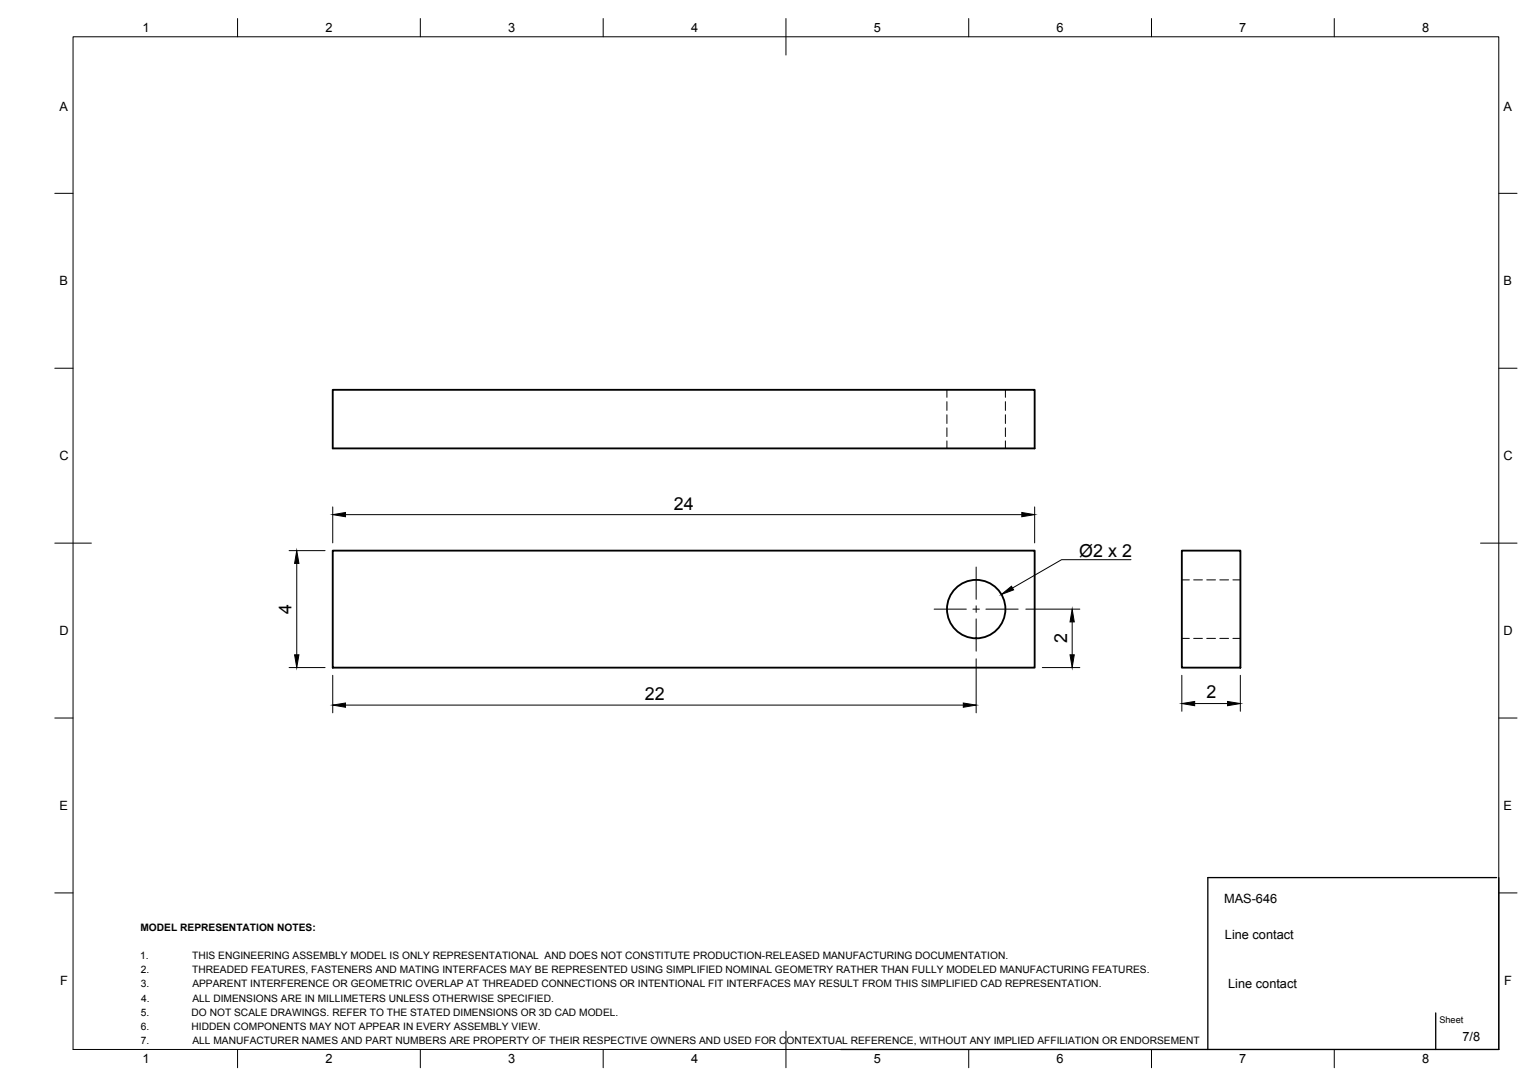
ISO-10303-21;
HEADER;
/* Generated by software containing ST-Developer
 * from STEP Tools, Inc. (www.steptools.com) 
 */

FILE_DESCRIPTION(
/* description */ ('Independent keyed three-contact power inlet for the IEC-connector des
ign category. Longer ground blade, retained contacts, wire termination
 holes and sealed bolted panel interface. Nominal custom interface; IE
C dimensional compatibility and electrical ratings are not assigned.'),

/* implementation_level */ '2;1');

FILE_NAME(
/* name */ 'Line contact.step',
/* time_stamp */ '2026-11-08T19:55:04-08:00',
/* author */ (''),
/* organization */ (''),
/* preprocessor_version */ 'ST-DEVELOPER v20.2',
/* originating_system */ 'Autodesk Translation Framework v15.17.0.0',
/* authorisation */ '');

FILE_SCHEMA (('AUTOMOTIVE_DESIGN { 1 0 10303 214 3 1 1 }'));
ENDSEC;

DATA;
#10=MECHANICAL_DESIGN_GEOMETRIC_PRESENTATION_REPRESENTATION('',(#114),#21880);
#94=SHAPE_REPRESENTATION_RELATIONSHIP('SRR','None',#21930,#104);
#104=ADVANCED_BREP_SHAPE_REPRESENTATION('',(#124),#21875);
#114=STYLED_ITEM('',(#21988),#124);
#124=MANIFOLD_SOLID_BREP('Body1',#6386);
#187=FACE_BOUND('',#944,.T.);
#188=FACE_BOUND('',#947,.T.);
#277=PLANE('',#6816);
#278=PLANE('',#6817);
#279=PLANE('',#6818);
#280=PLANE('',#6819);
#281=PLANE('',#6820);
#282=PLANE('',#6821);
#554=FACE_OUTER_BOUND('',#942,.T.);
#555=FACE_OUTER_BOUND('',#943,.T.);
#556=FACE_OUTER_BOUND('',#945,.T.);
#557=FACE_OUTER_BOUND('',#946,.T.);
#558=FACE_OUTER_BOUND('',#948,.T.);
#559=FACE_OUTER_BOUND('',#949,.T.);
#560=FACE_OUTER_BOUND('',#950,.T.);
#942=EDGE_LOOP('',(#5225,#5226,#5227,#5228));
#943=EDGE_LOOP('',(#5229,#5230,#5231,#5232));
#944=EDGE_LOOP('',(#5233));
#945=EDGE_LOOP('',(#5234,#5235,#5236,#5237));
#946=EDGE_LOOP('',(#5238,#5239,#5240,#5241));
#947=EDGE_LOOP('',(#5242));
#948=EDGE_LOOP('',(#5243,#5244,#5245,#5246));
#949=EDGE_LOOP('',(#5247,#5248,#5249,#5250));
#950=EDGE_LOOP('',(#5251,#5252,#5253,#5254));
#1138=CIRCLE('',#6814,1.);
#1139=CIRCLE('',#6815,1.);
#1852=LINE('',#16319,#2308);
#1853=LINE('',#16324,#2309);
#1854=LINE('',#16326,#2310);
#1855=LINE('',#16328,#2311);
#1856=LINE('',#16329,#2312);
#1857=LINE('',#16332,#2313);
#1858=LINE('',#16334,#2314);
#1859=LINE('',#16335,#2315);
#1860=LINE('',#16338,#2316);
#1861=LINE('',#16340,#2317);
#1862=LINE('',#16341,#2318);
#1863=LINE('',#16343,#2319);
#1864=LINE('',#16344,#2320);
#2308=VECTOR('',#7916,1.);
#2309=VECTOR('',#7921,10.);
#2310=VECTOR('',#7922,10.);
#2311=VECTOR('',#7923,10.);
#2312=VECTOR('',#7924,10.);
#2313=VECTOR('',#7927,10.);
#2314=VECTOR('',#7928,10.);
#2315=VECTOR('',#7929,10.);
#2316=VECTOR('',#7932,10.);
#2317=VECTOR('',#7933,10.);
#2318=VECTOR('',#7934,10.);
#2319=VECTOR('',#7937,10.);
#2320=VECTOR('',#7938,10.);
#2845=VERTEX_POINT('',#16316);
#2846=VERTEX_POINT('',#16318);
#2847=VERTEX_POINT('',#16322);
#2848=VERTEX_POINT('',#16323);
#2849=VERTEX_POINT('',#16325);
#2850=VERTEX_POINT('',#16327);
#2851=VERTEX_POINT('',#16331);
#2852=VERTEX_POINT('',#16333);
#2853=VERTEX_POINT('',#16337);
#2854=VERTEX_POINT('',#16339);
#3672=EDGE_CURVE('',#2845,#2845,#1138,.T.);
#3673=EDGE_CURVE('',#2845,#2846,#1852,.T.);
#3674=EDGE_CURVE('',#2846,#2846,#1139,.T.);
#3675=EDGE_CURVE('',#2847,#2848,#1853,.T.);
#3676=EDGE_CURVE('',#2848,#2849,#1854,.T.);
#3677=EDGE_CURVE('',#2850,#2849,#1855,.T.);
#3678=EDGE_CURVE('',#2847,#2850,#1856,.T.);
#3679=EDGE_CURVE('',#2851,#2847,#1857,.T.);
#3680=EDGE_CURVE('',#2852,#2850,#1858,.T.);
#3681=EDGE_CURVE('',#2851,#2852,#1859,.T.);
#3682=EDGE_CURVE('',#2853,#2851,#1860,.T.);
#3683=EDGE_CURVE('',#2854,#2852,#1861,.T.);
#3684=EDGE_CURVE('',#2853,#2854,#1862,.T.);
#3685=EDGE_CURVE('',#2848,#2853,#1863,.T.);
#3686=EDGE_CURVE('',#2849,#2854,#1864,.T.);
#5225=ORIENTED_EDGE('',*,*,#3672,.F.);
#5226=ORIENTED_EDGE('',*,*,#3673,.T.);
#5227=ORIENTED_EDGE('',*,*,#3674,.F.);
#5228=ORIENTED_EDGE('',*,*,#3673,.F.);
#5229=ORIENTED_EDGE('',*,*,#3675,.T.);
#5230=ORIENTED_EDGE('',*,*,#3676,.T.);
#5231=ORIENTED_EDGE('',*,*,#3677,.F.);
#5232=ORIENTED_EDGE('',*,*,#3678,.F.);
#5233=ORIENTED_EDGE('',*,*,#3672,.T.);
#5234=ORIENTED_EDGE('',*,*,#3679,.T.);
#5235=ORIENTED_EDGE('',*,*,#3678,.T.);
#5236=ORIENTED_EDGE('',*,*,#3680,.F.);
#5237=ORIENTED_EDGE('',*,*,#3681,.F.);
#5238=ORIENTED_EDGE('',*,*,#3682,.T.);
#5239=ORIENTED_EDGE('',*,*,#3681,.T.);
#5240=ORIENTED_EDGE('',*,*,#3683,.F.);
#5241=ORIENTED_EDGE('',*,*,#3684,.F.);
#5242=ORIENTED_EDGE('',*,*,#3674,.T.);
#5243=ORIENTED_EDGE('',*,*,#3685,.T.);
#5244=ORIENTED_EDGE('',*,*,#3684,.T.);
#5245=ORIENTED_EDGE('',*,*,#3686,.F.);
#5246=ORIENTED_EDGE('',*,*,#3676,.F.);
#5247=ORIENTED_EDGE('',*,*,#3686,.T.);
#5248=ORIENTED_EDGE('',*,*,#3683,.T.);
#5249=ORIENTED_EDGE('',*,*,#3680,.T.);
#5250=ORIENTED_EDGE('',*,*,#3677,.T.);
#5251=ORIENTED_EDGE('',*,*,#3685,.F.);
#5252=ORIENTED_EDGE('',*,*,#3675,.F.);
#5253=ORIENTED_EDGE('',*,*,#3679,.F.);
#5254=ORIENTED_EDGE('',*,*,#3682,.F.);
#5964=CYLINDRICAL_SURFACE('',#6813,1.);
#6266=ADVANCED_FACE('',(#554),#5964,.F.);
#6267=ADVANCED_FACE('',(#555,#187),#277,.T.);
#6268=ADVANCED_FACE('',(#556),#278,.T.);
#6269=ADVANCED_FACE('',(#557,#188),#279,.T.);
#6270=ADVANCED_FACE('',(#558),#280,.T.);
#6271=ADVANCED_FACE('',(#559),#281,.T.);
#6272=ADVANCED_FACE('',(#560),#282,.F.);
#6386=CLOSED_SHELL('',(#6266,#6267,#6268,#6269,#6270,#6271,#6272));
#6812=AXIS2_PLACEMENT_3D('',#16314,#7910,#7911);
#6813=AXIS2_PLACEMENT_3D('',#16315,#7912,#7913);
#6814=AXIS2_PLACEMENT_3D('',#16317,#7914,#7915);
#6815=AXIS2_PLACEMENT_3D('',#16320,#7917,#7918);
#6816=AXIS2_PLACEMENT_3D('',#16321,#7919,#7920);
#6817=AXIS2_PLACEMENT_3D('',#16330,#7925,#7926);
#6818=AXIS2_PLACEMENT_3D('',#16336,#7930,#7931);
#6819=AXIS2_PLACEMENT_3D('',#16342,#7935,#7936);
#6820=AXIS2_PLACEMENT_3D('',#16345,#7939,#7940);
#6821=AXIS2_PLACEMENT_3D('',#16346,#7941,#7942);
#7910=DIRECTION('axis',(0.,0.,1.));
#7911=DIRECTION('refdir',(1.,0.,0.));
#7912=DIRECTION('center_axis',(0.,-1.,0.));
#7913=DIRECTION('ref_axis',(0.,0.,1.));
#7914=DIRECTION('center_axis',(0.,-1.,0.));
#7915=DIRECTION('ref_axis',(0.,0.,1.));
#7916=DIRECTION('',(0.,-1.,0.));
#7917=DIRECTION('center_axis',(0.,1.,0.));
#7918=DIRECTION('ref_axis',(0.,0.,1.));
#7919=DIRECTION('center_axis',(0.,1.,0.));
#7920=DIRECTION('ref_axis',(-1.,0.,0.));
#7921=DIRECTION('',(-1.,0.,0.));
#7922=DIRECTION('',(0.,0.,1.));
#7923=DIRECTION('',(-1.,0.,0.));
#7924=DIRECTION('',(0.,0.,1.));
#7925=DIRECTION('center_axis',(1.,0.,0.));
#7926=DIRECTION('ref_axis',(0.,1.,0.));
#7927=DIRECTION('',(0.,1.,0.));
#7928=DIRECTION('',(0.,1.,0.));
#7929=DIRECTION('',(0.,0.,1.));
#7930=DIRECTION('center_axis',(0.,-1.,0.));
#7931=DIRECTION('ref_axis',(1.,0.,0.));
#7932=DIRECTION('',(1.,0.,0.));
#7933=DIRECTION('',(1.,0.,0.));
#7934=DIRECTION('',(0.,0.,1.));
#7935=DIRECTION('center_axis',(-1.,0.,0.));
#7936=DIRECTION('ref_axis',(0.,-1.,0.));
#7937=DIRECTION('',(0.,-1.,0.));
#7938=DIRECTION('',(0.,-1.,0.));
#7939=DIRECTION('center_axis',(0.,0.,1.));
#7940=DIRECTION('ref_axis',(1.,0.,0.));
#7941=DIRECTION('center_axis',(0.,0.,1.));
#7942=DIRECTION('ref_axis',(1.,0.,0.));
#16314=CARTESIAN_POINT('',(0.,0.,0.));
#16315=CARTESIAN_POINT('Origin',(0.,0.,2.));
#16316=CARTESIAN_POINT('',(1.22464679914735E-16,1.,1.));
#16317=CARTESIAN_POINT('Origin',(0.,1.,2.));
#16318=CARTESIAN_POINT('',(1.22464679914735E-16,-1.,1.));
#16319=CARTESIAN_POINT('',(1.22464679914735E-16,0.,1.));
#16320=CARTESIAN_POINT('Origin',(0.,-1.,2.));
#16321=CARTESIAN_POINT('Origin',(2.,1.,0.));
#16322=CARTESIAN_POINT('',(2.,1.,0.));
#16323=CARTESIAN_POINT('',(-2.,1.,0.));
#16324=CARTESIAN_POINT('',(2.,1.,0.));
#16325=CARTESIAN_POINT('',(-2.,1.,24.));
#16326=CARTESIAN_POINT('',(-2.,1.,0.));
#16327=CARTESIAN_POINT('',(2.,1.,24.));
#16328=CARTESIAN_POINT('',(2.,1.,24.));
#16329=CARTESIAN_POINT('',(2.,1.,0.));
#16330=CARTESIAN_POINT('Origin',(2.,-1.,0.));
#16331=CARTESIAN_POINT('',(2.,-1.,0.));
#16332=CARTESIAN_POINT('',(2.,-1.,0.));
#16333=CARTESIAN_POINT('',(2.,-1.,24.));
#16334=CARTESIAN_POINT('',(2.,-1.,24.));
#16335=CARTESIAN_POINT('',(2.,-1.,0.));
#16336=CARTESIAN_POINT('Origin',(-2.,-1.,0.));
#16337=CARTESIAN_POINT('',(-2.,-1.,0.));
#16338=CARTESIAN_POINT('',(-2.,-1.,0.));
#16339=CARTESIAN_POINT('',(-2.,-1.,24.));
#16340=CARTESIAN_POINT('',(-2.,-1.,24.));
#16341=CARTESIAN_POINT('',(-2.,-1.,0.));
#16342=CARTESIAN_POINT('Origin',(-2.,1.,0.));
#16343=CARTESIAN_POINT('',(-2.,1.,0.));
#16344=CARTESIAN_POINT('',(-2.,1.,24.));
#16345=CARTESIAN_POINT('Origin',(0.,0.,24.));
#16346=CARTESIAN_POINT('Origin',(0.,0.,0.));
#21863=UNCERTAINTY_MEASURE_WITH_UNIT(LENGTH_MEASURE(0.01),#21881,
'DISTANCE_ACCURACY_VALUE',
'Maximum model space distance between geometric entities at asserted c
onnectivities');
#21868=UNCERTAINTY_MEASURE_WITH_UNIT(LENGTH_MEASURE(0.01),#21881,
'DISTANCE_ACCURACY_VALUE',
'Maximum model space distance between geometric entities at asserted c
onnectivities');
#21875=(
GEOMETRIC_REPRESENTATION_CONTEXT(3)
GLOBAL_UNCERTAINTY_ASSIGNED_CONTEXT((#21863))
GLOBAL_UNIT_ASSIGNED_CONTEXT((#21881,#21883,#21884))
REPRESENTATION_CONTEXT('','3D')
);
#21880=(
GEOMETRIC_REPRESENTATION_CONTEXT(3)
GLOBAL_UNCERTAINTY_ASSIGNED_CONTEXT((#21868))
GLOBAL_UNIT_ASSIGNED_CONTEXT((#21881,#21883,#21884))
REPRESENTATION_CONTEXT('','3D')
);
#21881=(
LENGTH_UNIT()
NAMED_UNIT(*)
SI_UNIT(.MILLI.,.METRE.)
);
#21883=(
NAMED_UNIT(*)
PLANE_ANGLE_UNIT()
SI_UNIT($,.RADIAN.)
);
#21884=(
NAMED_UNIT(*)
SI_UNIT($,.STERADIAN.)
SOLID_ANGLE_UNIT()
);
#21891=SHAPE_DEFINITION_REPRESENTATION(#21902,#21930);
#21902=PRODUCT_DEFINITION_SHAPE('',$,#21942);
#21930=SHAPE_REPRESENTATION('',(#6812),#21875);
#21935=PRODUCT_DEFINITION_CONTEXT('part definition',#21970,'design');
#21942=PRODUCT_DEFINITION('Line contact','Line contact',#21953,#21935);
#21953=PRODUCT_DEFINITION_FORMATION('',$,#21978);
#21970=APPLICATION_CONTEXT(
'Core Data for Automotive Mechanical Design Process');
#21971=PRODUCT_CONTEXT('part definition',#21970,'mechanical');
#21978=PRODUCT('Line contact','Line contact',$,(#21971));
#21988=PRESENTATION_STYLE_ASSIGNMENT((#21994));
#21994=SURFACE_STYLE_USAGE(.BOTH.,#22000);
#22000=SURFACE_SIDE_STYLE('',(#22006));
#22006=SURFACE_STYLE_FILL_AREA(#22012);
#22012=FILL_AREA_STYLE('Light gray',(#22018));
#22018=FILL_AREA_STYLE_COLOUR('Light gray',#22024);
#22024=COLOUR_RGB('Light gray',0.725490196078431,0.752941176470588,0.792156862745098);
ENDSEC;
END-ISO-10303-21;
